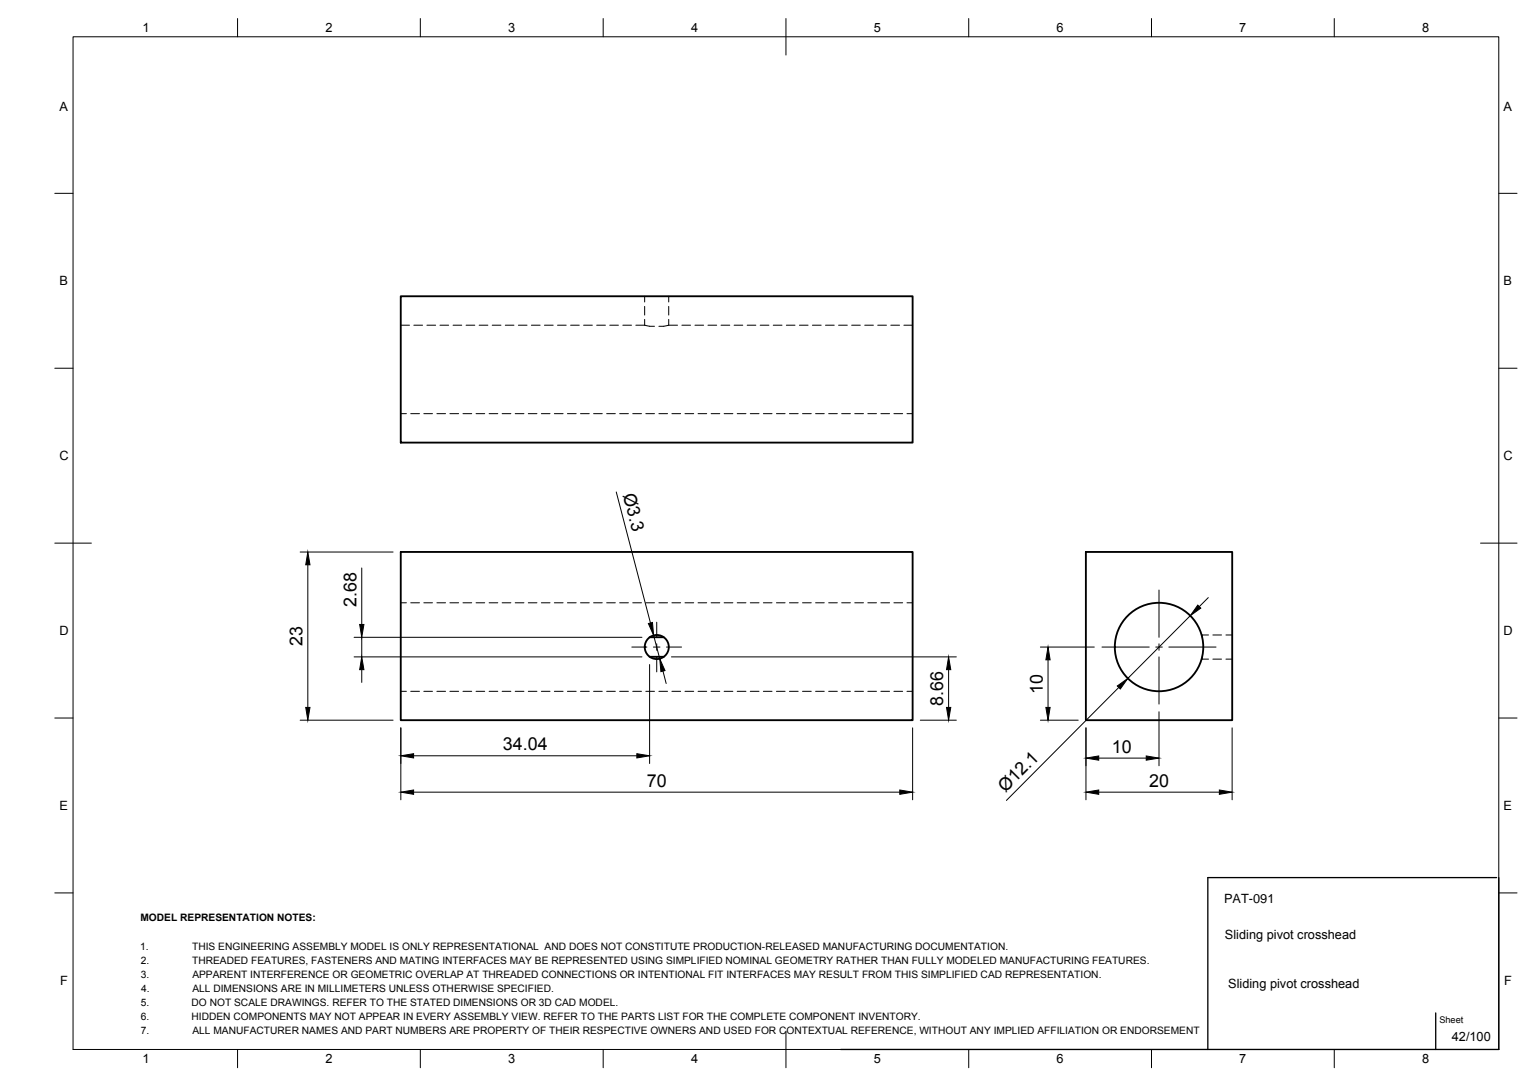
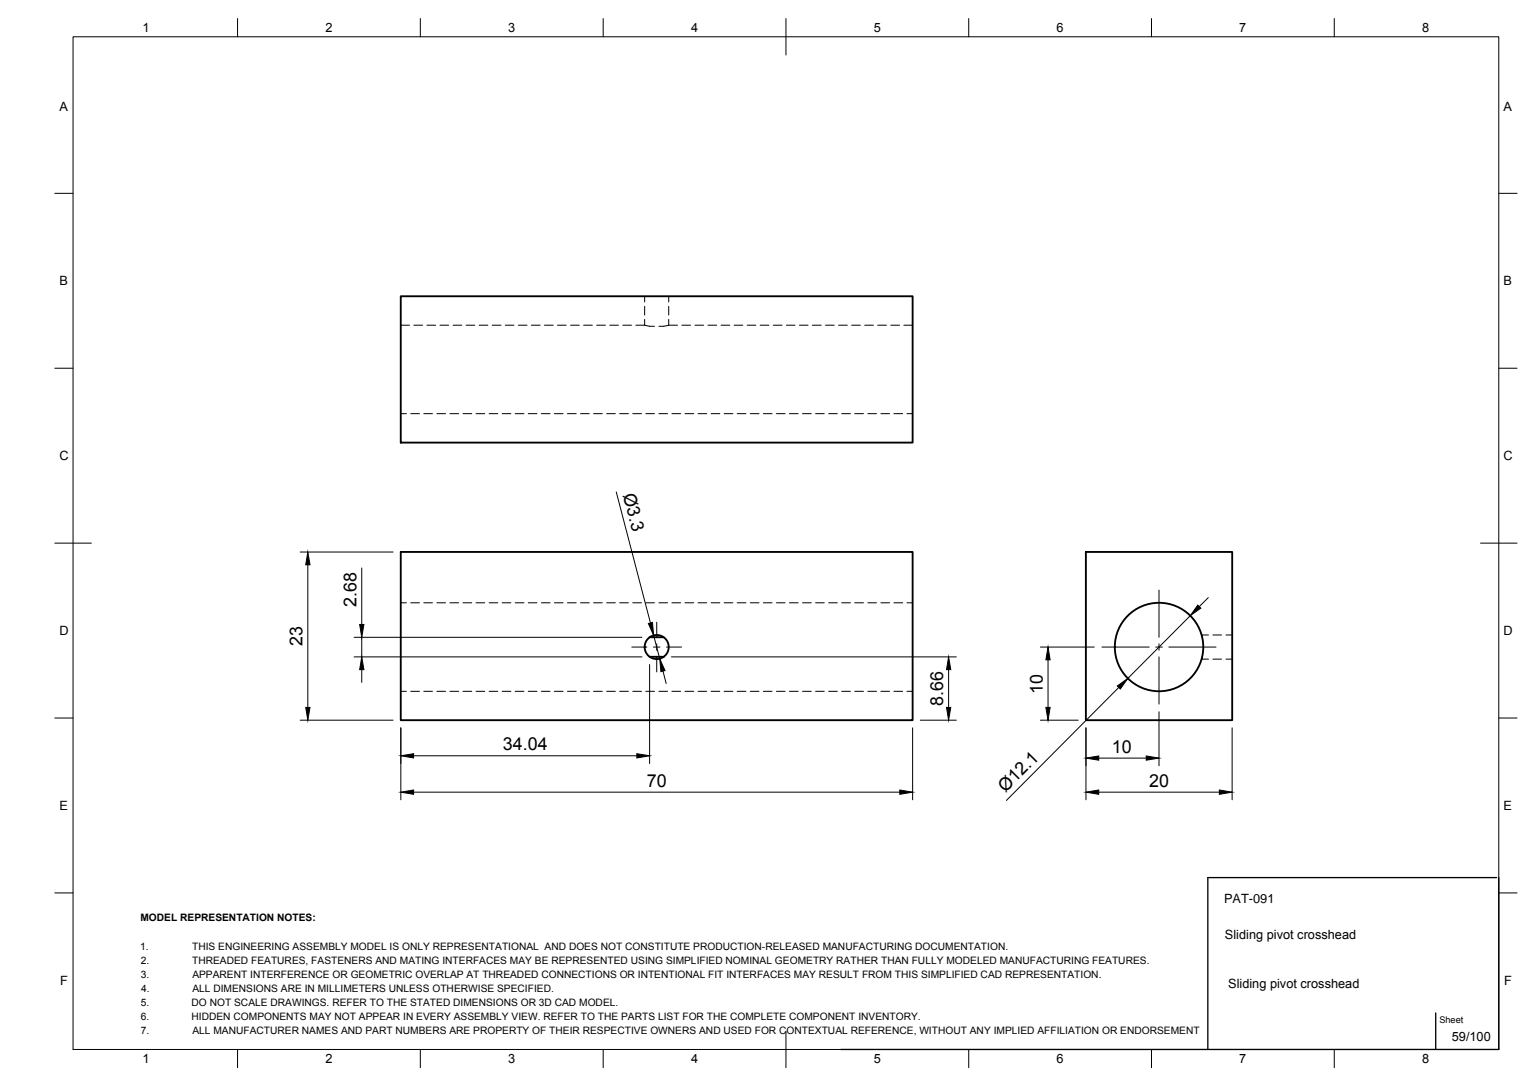
ISO-10303-21;
HEADER;
/* Generated by software containing ST-Developer
 * from STEP Tools, Inc. (www.steptools.com) 
 */

FILE_DESCRIPTION(
/* description */ ('PAT-091'),
/* implementation_level */ '2;1');

FILE_NAME(
/* name */ 'Sliding pivot crosshead.step',
/* time_stamp */ '2026-10-27T15:34:44-07:00',
/* author */ (''),
/* organization */ (''),
/* preprocessor_version */ 'ST-DEVELOPER v20.2',
/* originating_system */ 'Autodesk Translation Framework v15.17.0.0',
/* authorisation */ '');

FILE_SCHEMA (('AUTOMOTIVE_DESIGN { 1 0 10303 214 3 1 1 }'));
ENDSEC;

DATA;
#10=MECHANICAL_DESIGN_GEOMETRIC_PRESENTATION_REPRESENTATION('',(#1005),#25100);
#697=B_SPLINE_CURVE_WITH_KNOTS('',3,(#22341,#22342,#22343,#22344,#22345,
#22346,#22347,#22348,#22349,#22350,#22351,#22352,#22353,#22354),
 .UNSPECIFIED.,.F.,.F.,(4,2,2,2,2,2,4),(0.598759558597954,0.624973342427791,
0.687463163426143,0.749952984424496,0.812442805422848,0.874932626421201,
0.901146410251039),.UNSPECIFIED.);
#698=B_SPLINE_CURVE_WITH_KNOTS('',3,(#22362,#22363,#22364,#22365,#22366,
#22367,#22368,#22369,#22370,#22371,#22372,#22373,#22374,#22375),
 .UNSPECIFIED.,.F.,.F.,(4,2,2,2,2,2,4),(0.0987909023149563,0.125004686144793,
0.187494507143146,0.249984328141499,0.312474149139851,0.374963970138204,
0.401177753968041),.UNSPECIFIED.);
#785=SHAPE_REPRESENTATION_RELATIONSHIP('SRR','None',#25548,#895);
#895=ADVANCED_BREP_SHAPE_REPRESENTATION('',(#1127),#25018);
#1005=STYLED_ITEM('',(#26205),#1127);
#1127=MANIFOLD_SOLID_BREP('Body1',#13284);
#1414=FACE_BOUND('',#3379,.T.);
#1415=FACE_BOUND('',#3381,.T.);
#1416=FACE_BOUND('',#3383,.T.);
#1417=FACE_BOUND('',#3385,.T.);
#1799=PLANE('',#15184);
#1800=PLANE('',#15190);
#1801=PLANE('',#15194);
#1802=PLANE('',#15195);
#1803=PLANE('',#15196);
#1804=PLANE('',#15197);
#1805=PLANE('',#15198);
#1806=PLANE('',#15199);
#2358=FACE_OUTER_BOUND('',#3375,.T.);
#2359=FACE_OUTER_BOUND('',#3376,.T.);
#2360=FACE_OUTER_BOUND('',#3377,.T.);
#2361=FACE_OUTER_BOUND('',#3378,.T.);
#2362=FACE_OUTER_BOUND('',#3380,.T.);
#2363=FACE_OUTER_BOUND('',#3382,.T.);
#2364=FACE_OUTER_BOUND('',#3384,.T.);
#2365=FACE_OUTER_BOUND('',#3386,.T.);
#2366=FACE_OUTER_BOUND('',#3387,.T.);
#2367=FACE_OUTER_BOUND('',#3388,.T.);
#3375=EDGE_LOOP('',(#10206,#10207));
#3376=EDGE_LOOP('',(#10208,#10209,#10210,#10211,#10212,#10213,#10214,#10215));
#3377=EDGE_LOOP('',(#10216,#10217,#10218));
#3378=EDGE_LOOP('',(#10219,#10220,#10221,#10222));
#3379=EDGE_LOOP('',(#10223,#10224,#10225,#10226));
#3380=EDGE_LOOP('',(#10227,#10228,#10229,#10230));
#3381=EDGE_LOOP('',(#10231));
#3382=EDGE_LOOP('',(#10232,#10233,#10234,#10235));
#3383=EDGE_LOOP('',(#10236));
#3384=EDGE_LOOP('',(#10237,#10238,#10239,#10240));
#3385=EDGE_LOOP('',(#10241));
#3386=EDGE_LOOP('',(#10242,#10243,#10244,#10245));
#3387=EDGE_LOOP('',(#10246,#10247,#10248,#10249));
#3388=EDGE_LOOP('',(#10250,#10251,#10252,#10253));
#4476=LINE('',#22337,#5216);
#4477=LINE('',#22358,#5217);
#4478=LINE('',#22377,#5218);
#4479=LINE('',#22382,#5219);
#4480=LINE('',#22387,#5220);
#4481=LINE('',#22389,#5221);
#4482=LINE('',#22391,#5222);
#4483=LINE('',#22392,#5223);
#4484=LINE('',#22395,#5224);
#4485=LINE('',#22397,#5225);
#4486=LINE('',#22398,#5226);
#4487=LINE('',#22401,#5227);
#4488=LINE('',#22403,#5228);
#4489=LINE('',#22404,#5229);
#4490=LINE('',#22406,#5230);
#4491=LINE('',#22407,#5231);
#5216=VECTOR('',#18020,1.);
#5217=VECTOR('',#18027,0.165);
#5218=VECTOR('',#18034,1.);
#5219=VECTOR('',#18039,0.604999999999997);
#5220=VECTOR('',#18044,1.);
#5221=VECTOR('',#18045,1.);
#5222=VECTOR('',#18046,1.);
#5223=VECTOR('',#18047,1.);
#5224=VECTOR('',#18050,1.);
#5225=VECTOR('',#18051,1.);
#5226=VECTOR('',#18052,1.);
#5227=VECTOR('',#18055,1.);
#5228=VECTOR('',#18056,1.);
#5229=VECTOR('',#18057,1.);
#5230=VECTOR('',#18060,1.);
#5231=VECTOR('',#18061,1.);
#5869=CIRCLE('',#15185,0.165);
#5870=CIRCLE('',#15187,0.165);
#5871=CIRCLE('',#15188,0.165);
#5872=CIRCLE('',#15189,0.165);
#5873=CIRCLE('',#15192,0.604999999999997);
#5874=CIRCLE('',#15193,0.604999999999997);
#6792=VERTEX_POINT('',#22335);
#6793=VERTEX_POINT('',#22336);
#6794=VERTEX_POINT('',#22340);
#6795=VERTEX_POINT('',#22355);
#6796=VERTEX_POINT('',#22357);
#6797=VERTEX_POINT('',#22360);
#6798=VERTEX_POINT('',#22379);
#6799=VERTEX_POINT('',#22381);
#6800=VERTEX_POINT('',#22385);
#6801=VERTEX_POINT('',#22386);
#6802=VERTEX_POINT('',#22388);
#6803=VERTEX_POINT('',#22390);
#6804=VERTEX_POINT('',#22394);
#6805=VERTEX_POINT('',#22396);
#6806=VERTEX_POINT('',#22400);
#6807=VERTEX_POINT('',#22402);
#8038=EDGE_CURVE('',#6792,#6793,#4476,.T.);
#8039=EDGE_CURVE('',#6792,#6793,#5869,.T.);
#8040=EDGE_CURVE('',#6794,#6792,#697,.T.);
#8041=EDGE_CURVE('',#6795,#6794,#5870,.T.);
#8042=EDGE_CURVE('',#6795,#6796,#4477,.T.);
#8043=EDGE_CURVE('',#6796,#6796,#5871,.T.);
#8044=EDGE_CURVE('',#6797,#6795,#5872,.T.);
#8045=EDGE_CURVE('',#6793,#6797,#698,.T.);
#8046=EDGE_CURVE('',#6797,#6794,#4478,.T.);
#8047=EDGE_CURVE('',#6798,#6798,#5873,.T.);
#8048=EDGE_CURVE('',#6798,#6799,#4479,.T.);
#8049=EDGE_CURVE('',#6799,#6799,#5874,.T.);
#8050=EDGE_CURVE('',#6800,#6801,#4480,.T.);
#8051=EDGE_CURVE('',#6801,#6802,#4481,.T.);
#8052=EDGE_CURVE('',#6803,#6802,#4482,.T.);
#8053=EDGE_CURVE('',#6800,#6803,#4483,.T.);
#8054=EDGE_CURVE('',#6804,#6800,#4484,.T.);
#8055=EDGE_CURVE('',#6805,#6803,#4485,.T.);
#8056=EDGE_CURVE('',#6804,#6805,#4486,.T.);
#8057=EDGE_CURVE('',#6806,#6804,#4487,.T.);
#8058=EDGE_CURVE('',#6807,#6805,#4488,.T.);
#8059=EDGE_CURVE('',#6806,#6807,#4489,.T.);
#8060=EDGE_CURVE('',#6801,#6806,#4490,.T.);
#8061=EDGE_CURVE('',#6802,#6807,#4491,.T.);
#10206=ORIENTED_EDGE('',*,*,#8038,.F.);
#10207=ORIENTED_EDGE('',*,*,#8039,.T.);
#10208=ORIENTED_EDGE('',*,*,#8040,.F.);
#10209=ORIENTED_EDGE('',*,*,#8041,.F.);
#10210=ORIENTED_EDGE('',*,*,#8042,.T.);
#10211=ORIENTED_EDGE('',*,*,#8043,.F.);
#10212=ORIENTED_EDGE('',*,*,#8042,.F.);
#10213=ORIENTED_EDGE('',*,*,#8044,.F.);
#10214=ORIENTED_EDGE('',*,*,#8045,.F.);
#10215=ORIENTED_EDGE('',*,*,#8039,.F.);
#10216=ORIENTED_EDGE('',*,*,#8046,.F.);
#10217=ORIENTED_EDGE('',*,*,#8044,.T.);
#10218=ORIENTED_EDGE('',*,*,#8041,.T.);
#10219=ORIENTED_EDGE('',*,*,#8047,.F.);
#10220=ORIENTED_EDGE('',*,*,#8048,.T.);
#10221=ORIENTED_EDGE('',*,*,#8049,.F.);
#10222=ORIENTED_EDGE('',*,*,#8048,.F.);
#10223=ORIENTED_EDGE('',*,*,#8045,.T.);
#10224=ORIENTED_EDGE('',*,*,#8046,.T.);
#10225=ORIENTED_EDGE('',*,*,#8040,.T.);
#10226=ORIENTED_EDGE('',*,*,#8038,.T.);
#10227=ORIENTED_EDGE('',*,*,#8050,.T.);
#10228=ORIENTED_EDGE('',*,*,#8051,.T.);
#10229=ORIENTED_EDGE('',*,*,#8052,.F.);
#10230=ORIENTED_EDGE('',*,*,#8053,.F.);
#10231=ORIENTED_EDGE('',*,*,#8049,.T.);
#10232=ORIENTED_EDGE('',*,*,#8054,.T.);
#10233=ORIENTED_EDGE('',*,*,#8053,.T.);
#10234=ORIENTED_EDGE('',*,*,#8055,.F.);
#10235=ORIENTED_EDGE('',*,*,#8056,.F.);
#10236=ORIENTED_EDGE('',*,*,#8043,.T.);
#10237=ORIENTED_EDGE('',*,*,#8057,.T.);
#10238=ORIENTED_EDGE('',*,*,#8056,.T.);
#10239=ORIENTED_EDGE('',*,*,#8058,.F.);
#10240=ORIENTED_EDGE('',*,*,#8059,.F.);
#10241=ORIENTED_EDGE('',*,*,#8047,.T.);
#10242=ORIENTED_EDGE('',*,*,#8060,.T.);
#10243=ORIENTED_EDGE('',*,*,#8059,.T.);
#10244=ORIENTED_EDGE('',*,*,#8061,.F.);
#10245=ORIENTED_EDGE('',*,*,#8051,.F.);
#10246=ORIENTED_EDGE('',*,*,#8061,.T.);
#10247=ORIENTED_EDGE('',*,*,#8058,.T.);
#10248=ORIENTED_EDGE('',*,*,#8055,.T.);
#10249=ORIENTED_EDGE('',*,*,#8052,.T.);
#10250=ORIENTED_EDGE('',*,*,#8060,.F.);
#10251=ORIENTED_EDGE('',*,*,#8050,.F.);
#10252=ORIENTED_EDGE('',*,*,#8054,.F.);
#10253=ORIENTED_EDGE('',*,*,#8057,.F.);
#12203=CYLINDRICAL_SURFACE('',#15186,0.165);
#12204=CYLINDRICAL_SURFACE('',#15191,0.604999999999997);
#12725=ADVANCED_FACE('',(#2358),#1799,.T.);
#12726=ADVANCED_FACE('',(#2359),#12203,.F.);
#12727=ADVANCED_FACE('',(#2360),#1800,.T.);
#12728=ADVANCED_FACE('',(#2361,#1414),#12204,.F.);
#12729=ADVANCED_FACE('',(#2362,#1415),#1801,.T.);
#12730=ADVANCED_FACE('',(#2363,#1416),#1802,.T.);
#12731=ADVANCED_FACE('',(#2364,#1417),#1803,.T.);
#12732=ADVANCED_FACE('',(#2365),#1804,.T.);
#12733=ADVANCED_FACE('',(#2366),#1805,.T.);
#12734=ADVANCED_FACE('',(#2367),#1806,.F.);
#13284=CLOSED_SHELL('',(#12725,#12726,#12727,#12728,#12729,#12730,#12731,
#12732,#12733,#12734));
#15183=AXIS2_PLACEMENT_3D('',#22333,#18016,#18017);
#15184=AXIS2_PLACEMENT_3D('',#22334,#18018,#18019);
#15185=AXIS2_PLACEMENT_3D('',#22338,#18021,#18022);
#15186=AXIS2_PLACEMENT_3D('',#22339,#18023,#18024);
#15187=AXIS2_PLACEMENT_3D('',#22356,#18025,#18026);
#15188=AXIS2_PLACEMENT_3D('',#22359,#18028,#18029);
#15189=AXIS2_PLACEMENT_3D('',#22361,#18030,#18031);
#15190=AXIS2_PLACEMENT_3D('',#22376,#18032,#18033);
#15191=AXIS2_PLACEMENT_3D('',#22378,#18035,#18036);
#15192=AXIS2_PLACEMENT_3D('',#22380,#18037,#18038);
#15193=AXIS2_PLACEMENT_3D('',#22383,#18040,#18041);
#15194=AXIS2_PLACEMENT_3D('',#22384,#18042,#18043);
#15195=AXIS2_PLACEMENT_3D('',#22393,#18048,#18049);
#15196=AXIS2_PLACEMENT_3D('',#22399,#18053,#18054);
#15197=AXIS2_PLACEMENT_3D('',#22405,#18058,#18059);
#15198=AXIS2_PLACEMENT_3D('',#22408,#18062,#18063);
#15199=AXIS2_PLACEMENT_3D('',#22409,#18064,#18065);
#18016=DIRECTION('axis',(0.,0.,1.));
#18017=DIRECTION('refdir',(1.,0.,0.));
#18018=DIRECTION('center_axis',(1.,0.,0.));
#18019=DIRECTION('ref_axis',(0.,0.,-1.));
#18020=DIRECTION('',(0.,1.,0.));
#18021=DIRECTION('center_axis',(1.,0.,0.));
#18022=DIRECTION('ref_axis',(0.,0.,-1.));
#18023=DIRECTION('center_axis',(1.,0.,0.));
#18024=DIRECTION('ref_axis',(0.,0.,-1.));
#18025=DIRECTION('center_axis',(1.,0.,0.));
#18026=DIRECTION('ref_axis',(0.,0.,-1.));
#18027=DIRECTION('',(1.,0.,0.));
#18028=DIRECTION('center_axis',(-1.,0.,0.));
#18029=DIRECTION('ref_axis',(0.,0.,-1.));
#18030=DIRECTION('center_axis',(1.,0.,0.));
#18031=DIRECTION('ref_axis',(0.,0.,-1.));
#18032=DIRECTION('center_axis',(1.,0.,0.));
#18033=DIRECTION('ref_axis',(0.,0.,-1.));
#18034=DIRECTION('',(0.,-1.,0.));
#18035=DIRECTION('center_axis',(0.,1.,0.));
#18036=DIRECTION('ref_axis',(1.,0.,0.));
#18037=DIRECTION('center_axis',(0.,1.,0.));
#18038=DIRECTION('ref_axis',(1.,0.,0.));
#18039=DIRECTION('',(0.,1.,0.));
#18040=DIRECTION('center_axis',(0.,-1.,0.));
#18041=DIRECTION('ref_axis',(1.,0.,0.));
#18042=DIRECTION('center_axis',(0.,1.,0.));
#18043=DIRECTION('ref_axis',(-1.,0.,0.));
#18044=DIRECTION('',(-1.,0.,0.));
#18045=DIRECTION('',(0.,0.,1.));
#18046=DIRECTION('',(-1.,0.,0.));
#18047=DIRECTION('',(0.,0.,1.));
#18048=DIRECTION('center_axis',(1.,0.,0.));
#18049=DIRECTION('ref_axis',(0.,1.,0.));
#18050=DIRECTION('',(0.,1.,0.));
#18051=DIRECTION('',(0.,1.,0.));
#18052=DIRECTION('',(0.,0.,1.));
#18053=DIRECTION('center_axis',(0.,-1.,0.));
#18054=DIRECTION('ref_axis',(1.,0.,0.));
#18055=DIRECTION('',(1.,0.,0.));
#18056=DIRECTION('',(1.,0.,0.));
#18057=DIRECTION('',(0.,0.,1.));
#18058=DIRECTION('center_axis',(-1.,0.,0.));
#18059=DIRECTION('ref_axis',(0.,-1.,0.));
#18060=DIRECTION('',(0.,-1.,0.));
#18061=DIRECTION('',(0.,-1.,0.));
#18062=DIRECTION('center_axis',(0.,0.,1.));
#18063=DIRECTION('ref_axis',(1.,0.,0.));
#18064=DIRECTION('center_axis',(0.,0.,1.));
#18065=DIRECTION('ref_axis',(1.,0.,0.));
#22333=CARTESIAN_POINT('',(0.,0.,0.));
#22334=CARTESIAN_POINT('Origin',(39.31983346,0.,3.));
#22335=CARTESIAN_POINT('',(39.31983346,-0.0964364949201869,2.86611571246965));
#22336=CARTESIAN_POINT('',(39.31983346,0.0964364949201869,2.86611571246965));
#22337=CARTESIAN_POINT('',(39.31983346,-3.6,2.86611571246965));
#22338=CARTESIAN_POINT('Origin',(39.31983346,0.,3.));
#22339=CARTESIAN_POINT('Origin',(39.31983346,0.,3.));
#22340=CARTESIAN_POINT('',(39.31983346,-0.0964364949201869,3.13388428753035));
#22341=CARTESIAN_POINT('Ctrl Pts',(39.31983346,-0.0964364949201871,3.13388428753035));
#22342=CARTESIAN_POINT('Ctrl Pts',(39.3210318640464,-0.103768349789617,
3.1286031720394));
#22343=CARTESIAN_POINT('Ctrl Pts',(39.3222741026686,-0.110552785281794,
3.12279245250977));
#22344=CARTESIAN_POINT('Ctrl Pts',(39.3263441031883,-0.131261405831701,
3.10208383195986));
#22345=CARTESIAN_POINT('Ctrl Pts',(39.3293775570573,-0.143943476007901,
3.08360021359466));
#22346=CARTESIAN_POINT('Ctrl Pts',(39.3336505364571,-0.160815615633796,
3.04297741500427));
#22347=CARTESIAN_POINT('Ctrl Pts',(39.3348334620742,-0.165,3.02082994033278));
#22348=CARTESIAN_POINT('Ctrl Pts',(39.3348334620742,-0.165,2.97917005966722));
#22349=CARTESIAN_POINT('Ctrl Pts',(39.3336505364571,-0.160815615633796,
2.95702258499573));
#22350=CARTESIAN_POINT('Ctrl Pts',(39.3293775570573,-0.143943476007901,
2.91639978640534));
#22351=CARTESIAN_POINT('Ctrl Pts',(39.3263441031883,-0.131261405831701,
2.89791616804014));
#22352=CARTESIAN_POINT('Ctrl Pts',(39.3222741026686,-0.110552785281793,
2.87720754749023));
#22353=CARTESIAN_POINT('Ctrl Pts',(39.3210318640464,-0.103768349789617,
2.8713968279606));
#22354=CARTESIAN_POINT('Ctrl Pts',(39.31983346,-0.0964364949201869,2.86611571246965));
#22355=CARTESIAN_POINT('',(39.31983346,-2.02066721859313E-17,3.165));
#22356=CARTESIAN_POINT('Origin',(39.31983346,0.,3.));
#22357=CARTESIAN_POINT('',(39.7298334620742,2.02066721859313E-17,3.165));
#22358=CARTESIAN_POINT('',(39.31983346,-2.02066721859313E-17,3.165));
#22359=CARTESIAN_POINT('Origin',(39.7298334620742,0.,3.));
#22360=CARTESIAN_POINT('',(39.31983346,0.0964364949201869,3.13388428753035));
#22361=CARTESIAN_POINT('Origin',(39.31983346,0.,3.));
#22362=CARTESIAN_POINT('Ctrl Pts',(39.31983346,0.0964364949201869,2.86611571246965));
#22363=CARTESIAN_POINT('Ctrl Pts',(39.3210318640464,0.103768349789617,2.8713968279606));
#22364=CARTESIAN_POINT('Ctrl Pts',(39.3222741026686,0.110552785281793,2.87720754749023));
#22365=CARTESIAN_POINT('Ctrl Pts',(39.3263441031883,0.1312614058317,2.89791616804014));
#22366=CARTESIAN_POINT('Ctrl Pts',(39.3293775570573,0.143943476007901,2.91639978640534));
#22367=CARTESIAN_POINT('Ctrl Pts',(39.3336505364571,0.160815615633796,2.95702258499573));
#22368=CARTESIAN_POINT('Ctrl Pts',(39.3348334620742,0.165,2.97917005966722));
#22369=CARTESIAN_POINT('Ctrl Pts',(39.3348334620742,0.165,3.02082994033278));
#22370=CARTESIAN_POINT('Ctrl Pts',(39.3336505364571,0.160815615633796,3.04297741500427));
#22371=CARTESIAN_POINT('Ctrl Pts',(39.3293775570573,0.143943476007901,3.08360021359466));
#22372=CARTESIAN_POINT('Ctrl Pts',(39.3263441031883,0.1312614058317,3.10208383195986));
#22373=CARTESIAN_POINT('Ctrl Pts',(39.3222741026686,0.110552785281793,3.12279245250977));
#22374=CARTESIAN_POINT('Ctrl Pts',(39.3210318640464,0.103768349789617,3.1286031720394));
#22375=CARTESIAN_POINT('Ctrl Pts',(39.31983346,0.0964364949201871,3.13388428753035));
#22376=CARTESIAN_POINT('Origin',(39.31983346,0.,3.));
#22377=CARTESIAN_POINT('',(39.31983346,-3.6,3.13388428753035));
#22378=CARTESIAN_POINT('Origin',(38.7298334620742,-3.6,3.));
#22379=CARTESIAN_POINT('',(38.1248334620742,-3.5,3.));
#22380=CARTESIAN_POINT('Origin',(38.7298334620742,-3.5,3.));
#22381=CARTESIAN_POINT('',(38.1248334620742,3.5,3.));
#22382=CARTESIAN_POINT('',(38.1248334620742,-3.6,3.));
#22383=CARTESIAN_POINT('Origin',(38.7298334620742,3.5,3.));
#22384=CARTESIAN_POINT('Origin',(39.7298334620742,3.5,2.));
#22385=CARTESIAN_POINT('',(39.7298334620742,3.5,2.));
#22386=CARTESIAN_POINT('',(37.7298334620742,3.5,2.));
#22387=CARTESIAN_POINT('',(39.7298334620742,3.5,2.));
#22388=CARTESIAN_POINT('',(37.7298334620742,3.5,4.3));
#22389=CARTESIAN_POINT('',(37.7298334620742,3.5,2.));
#22390=CARTESIAN_POINT('',(39.7298334620742,3.5,4.3));
#22391=CARTESIAN_POINT('',(39.7298334620742,3.5,4.3));
#22392=CARTESIAN_POINT('',(39.7298334620742,3.5,2.));
#22393=CARTESIAN_POINT('Origin',(39.7298334620742,-3.5,2.));
#22394=CARTESIAN_POINT('',(39.7298334620742,-3.5,2.));
#22395=CARTESIAN_POINT('',(39.7298334620742,-3.5,2.));
#22396=CARTESIAN_POINT('',(39.7298334620742,-3.5,4.3));
#22397=CARTESIAN_POINT('',(39.7298334620742,-3.5,4.3));
#22398=CARTESIAN_POINT('',(39.7298334620742,-3.5,2.));
#22399=CARTESIAN_POINT('Origin',(37.7298334620742,-3.5,2.));
#22400=CARTESIAN_POINT('',(37.7298334620742,-3.5,2.));
#22401=CARTESIAN_POINT('',(37.7298334620742,-3.5,2.));
#22402=CARTESIAN_POINT('',(37.7298334620742,-3.5,4.3));
#22403=CARTESIAN_POINT('',(37.7298334620742,-3.5,4.3));
#22404=CARTESIAN_POINT('',(37.7298334620742,-3.5,2.));
#22405=CARTESIAN_POINT('Origin',(37.7298334620742,3.5,2.));
#22406=CARTESIAN_POINT('',(37.7298334620742,3.5,2.));
#22407=CARTESIAN_POINT('',(37.7298334620742,3.5,4.3));
#22408=CARTESIAN_POINT('Origin',(38.7298334620742,0.,4.3));
#22409=CARTESIAN_POINT('Origin',(38.7298334620742,0.,2.));
#24897=UNCERTAINTY_MEASURE_WITH_UNIT(LENGTH_MEASURE(0.001),#25101,
'DISTANCE_ACCURACY_VALUE',
'Maximum model space distance between geometric entities at asserted c
onnectivities');
#24979=UNCERTAINTY_MEASURE_WITH_UNIT(LENGTH_MEASURE(0.001),#25101,
'DISTANCE_ACCURACY_VALUE',
'Maximum model space distance between geometric entities at asserted c
onnectivities');
#25018=(
GEOMETRIC_REPRESENTATION_CONTEXT(3)
GLOBAL_UNCERTAINTY_ASSIGNED_CONTEXT((#24897))
GLOBAL_UNIT_ASSIGNED_CONTEXT((#25101,#25103,#25104))
REPRESENTATION_CONTEXT('','3D')
);
#25100=(
GEOMETRIC_REPRESENTATION_CONTEXT(3)
GLOBAL_UNCERTAINTY_ASSIGNED_CONTEXT((#24979))
GLOBAL_UNIT_ASSIGNED_CONTEXT((#25101,#25103,#25104))
REPRESENTATION_CONTEXT('','3D')
);
#25101=(
LENGTH_UNIT()
NAMED_UNIT(*)
SI_UNIT(.CENTI.,.METRE.)
);
#25103=(
NAMED_UNIT(*)
PLANE_ANGLE_UNIT()
SI_UNIT($,.RADIAN.)
);
#25104=(
NAMED_UNIT(*)
SI_UNIT($,.STERADIAN.)
SOLID_ANGLE_UNIT()
);
#25143=SHAPE_DEFINITION_REPRESENTATION(#25263,#25548);
#25263=PRODUCT_DEFINITION_SHAPE('',$,#25669);
#25548=SHAPE_REPRESENTATION('',(#15183),#25018);
#25630=PRODUCT_DEFINITION_CONTEXT('part definition',#25992,'design');
#25669=PRODUCT_DEFINITION('Sliding pivot crosshead',
'Sliding pivot crosshead',#25789,#25630);
#25789=PRODUCT_DEFINITION_FORMATION('',$,#26032);
#25992=APPLICATION_CONTEXT(
'Core Data for Automotive Mechanical Design Process');
#25993=PRODUCT_CONTEXT('part definition',#25992,'mechanical');
#26032=PRODUCT('Sliding pivot crosshead','Sliding pivot crosshead',
'Sliding pivot crosshead',(#25993));
#26199=COLOUR_RGB('Off White',0.89,0.88,0.83);
#26200=FILL_AREA_STYLE_COLOUR('',#26199);
#26201=FILL_AREA_STYLE('',(#26200));
#26202=SURFACE_STYLE_FILL_AREA(#26201);
#26203=SURFACE_SIDE_STYLE('',(#26202));
#26204=SURFACE_STYLE_USAGE(.BOTH.,#26203);
#26205=PRESENTATION_STYLE_ASSIGNMENT((#26204));
ENDSEC;
END-ISO-10303-21;
